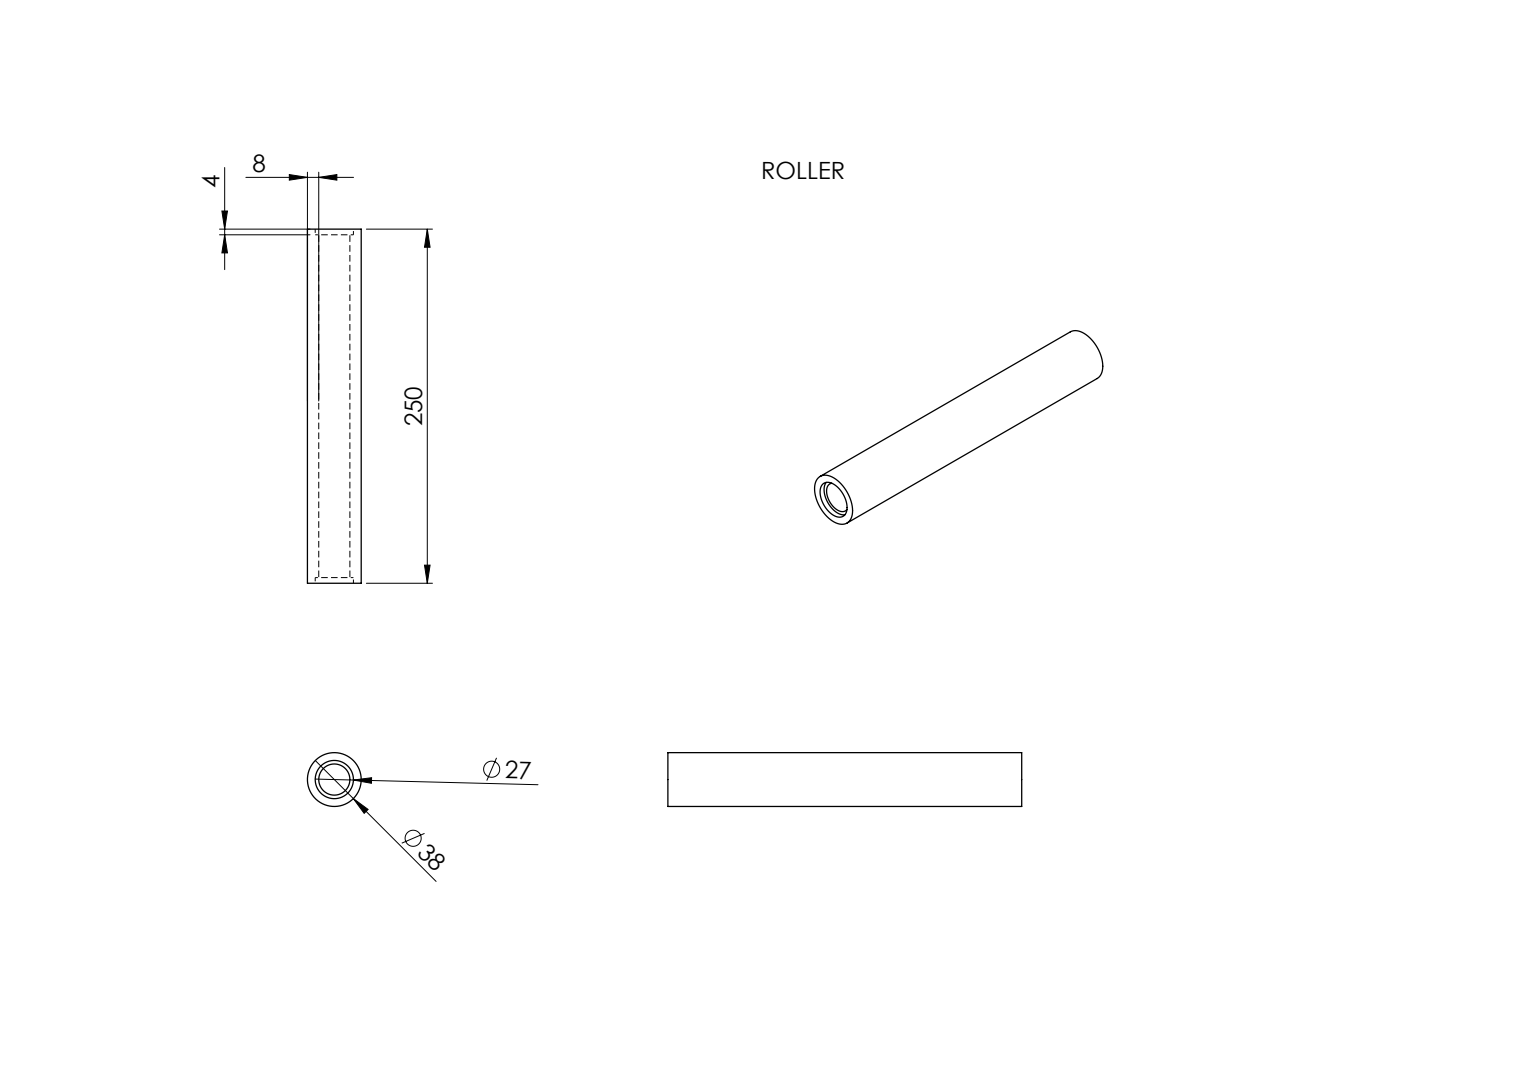
ISO-10303-21;
HEADER;
FILE_DESCRIPTION (('STEP AP214'),
    '1' );
FILE_NAME ('roller.step',
    '2026-10-24T14:05:44',
    ( '' ),
    ( '' ),
    'SwSTEP 2.0',
    'SolidWorks 2026',
    '' );
FILE_SCHEMA (( 'AUTOMOTIVE_DESIGN' ));
ENDSEC;

DATA;
#78=ADVANCED_FACE ( 'NONE', ( #707 ), #151, .F. ) ;
#101=CARTESIAN_POINT ( 'NONE',  ( 11.00000000000000000, 1.347111479062088405E-15, 121.0000000000000000 ) ) ;
#129=DIRECTION ( 'NONE',  ( 0.000000000000000000, 0.000000000000000000, 1.000000000000000000 ) ) ;
#130=DIRECTION ( 'NONE',  ( 0.000000000000000000, 0.000000000000000000, 1.000000000000000000 ) ) ;
#141=SURFACE_STYLE_USAGE ( .BOTH. , #4095 ) ;
#145=ADVANCED_FACE ( 'NONE', ( #6026 ), #5486, .F. ) ;
#151=CYLINDRICAL_SURFACE ( 'NONE', #6391, 13.50000000000000000 ) ;
#167=PLANE ( 'NONE',  #1333 ) ;
#204=ORIENTED_EDGE ( 'NONE', *, *, #2954, .T. ) ;
#232=EDGE_LOOP ( 'NONE', ( #859, #5751, #5107, #3402 ) ) ;
#286=EDGE_CURVE ( 'NONE', #7309, #3129, #6272, .T. ) ;
#299=CARTESIAN_POINT ( 'NONE',  ( 0.000000000000000000, 0.000000000000000000, 125.0000000000000000 ) ) ;
#385=DIRECTION ( 'NONE',  ( -0.000000000000000000, -0.000000000000000000, 1.000000000000000000 ) ) ;
#402=ADVANCED_BREP_SHAPE_REPRESENTATION ( '', ( #3126, #1963 ), #3131 ) ;
#447=AXIS2_PLACEMENT_3D ( 'NONE', #2275, #5736, #5768 ) ;
#495=CARTESIAN_POINT ( 'NONE',  ( 0.000000000000000000, 0.000000000000000000, -121.0000000000000000 ) ) ;
#501=EDGE_LOOP ( 'NONE', ( #2407, #5320, #3926, #4754 ) ) ;
#548=ORIENTED_EDGE ( 'NONE', *, *, #7125, .F. ) ;
#563=VERTEX_POINT ( 'NONE', #6568 ) ;
#566=CARTESIAN_POINT ( 'NONE',  ( -11.00000000000000000, 0.000000000000000000, 121.0000000000000000 ) ) ;
#628=DIRECTION ( 'NONE',  ( 0.000000000000000000, 0.000000000000000000, 1.000000000000000000 ) ) ;
#632=CIRCLE ( 'NONE', #7087, 19.00000000000000000 ) ;
#661=AXIS2_PLACEMENT_3D ( 'NONE', #7149, #4263, #2002 ) ;
#679=EDGE_LOOP ( 'NONE', ( #1531, #1316, #1080, #4303 ) ) ;
#681=DIRECTION ( 'NONE',  ( 1.000000000000000000, 0.000000000000000000, 0.000000000000000000 ) ) ;
#707=FACE_OUTER_BOUND ( 'NONE', #3501, .T. ) ;
#714=CARTESIAN_POINT ( 'NONE',  ( 0.000000000000000000, 0.000000000000000000, -121.0000000000000000 ) ) ;
#725=VECTOR ( 'NONE', #6797, 1000.000000000000000 ) ;
#761=ORIENTED_EDGE ( 'NONE', *, *, #5228, .T. ) ;
#764=AXIS2_PLACEMENT_3D ( 'NONE', #2213, #6804, #3945 ) ;
#780=AXIS2_PLACEMENT_3D ( 'NONE', #2339, #3531, #2993 ) ;
#787=DIRECTION ( 'NONE',  ( 1.000000000000000000, 0.000000000000000000, 0.000000000000000000 ) ) ;
#821=CARTESIAN_POINT ( 'NONE',  ( 0.000000000000000000, 0.000000000000000000, 125.0000000000000000 ) ) ;
#830=FACE_OUTER_BOUND ( 'NONE', #3358, .T. ) ;
#836=DIRECTION ( 'NONE',  ( -1.000000000000000000, 0.000000000000000000, 0.000000000000000000 ) ) ;
#859=ORIENTED_EDGE ( 'NONE', *, *, #4888, .F. ) ;
#866=AXIS2_PLACEMENT_3D ( 'NONE', #939, #3814, #4267 ) ;
#869=ORIENTED_EDGE ( 'NONE', *, *, #7028, .F. ) ;
#871=LINE ( 'NONE', #916, #4310 ) ;
#890=DIRECTION ( 'NONE',  ( -0.000000000000000000, -0.000000000000000000, -1.000000000000000000 ) ) ;
#902=ADVANCED_FACE ( 'NONE', ( #7143 ), #5410, .F. ) ;
#916=CARTESIAN_POINT ( 'NONE',  ( 13.50000000000000000, 1.653273178848926867E-15, -121.0000000000000000 ) ) ;
#921=AXIS2_PLACEMENT_3D ( 'NONE', #299, #2557, #3103 ) ;
#926=EDGE_CURVE ( 'NONE', #5946, #2821, #3721, .T. ) ;
#939=CARTESIAN_POINT ( 'NONE',  ( 0.000000000000000000, 0.000000000000000000, 125.0000000000000000 ) ) ;
#967=DIRECTION ( 'NONE',  ( 1.000000000000000000, 0.000000000000000000, 0.000000000000000000 ) ) ;
#993=DIRECTION ( 'NONE',  ( 0.000000000000000000, 0.000000000000000000, 1.000000000000000000 ) ) ;
#1017=DIRECTION ( 'NONE',  ( -0.000000000000000000, -0.000000000000000000, 1.000000000000000000 ) ) ;
#1022=CIRCLE ( 'NONE', #661, 11.00000000000000000 ) ;
#1027=PLANE ( 'NONE',  #4902 ) ;
#1029=CIRCLE ( 'NONE', #780, 19.00000000000000000 ) ;
#1044=ORIENTED_EDGE ( 'NONE', *, *, #286, .F. ) ;
#1063=DIRECTION ( 'NONE',  ( 1.000000000000000000, 0.000000000000000000, -0.000000000000000000 ) ) ;
#1069=CYLINDRICAL_SURFACE ( 'NONE', #764, 19.00000000000000000 ) ;
#1080=ORIENTED_EDGE ( 'NONE', *, *, #7028, .T. ) ;
#1133=CARTESIAN_POINT ( 'NONE',  ( 0.000000000000000000, 0.000000000000000000, 121.0000000000000000 ) ) ;
#1190=( NAMED_UNIT ( * ) PLANE_ANGLE_UNIT ( ) SI_UNIT ( $, .RADIAN. ) );
#1218=SHAPE_DEFINITION_REPRESENTATION ( #4339, #6025 ) ;
#1242=LINE ( 'NONE', #3584, #6951 ) ;
#1270=VECTOR ( 'NONE', #890, 1000.000000000000000 ) ;
#1277=FACE_OUTER_BOUND ( 'NONE', #3592, .T. ) ;
#1304=VERTEX_POINT ( 'NONE', #3677 ) ;
#1316=ORIENTED_EDGE ( 'NONE', *, *, #3473, .T. ) ;
#1333=AXIS2_PLACEMENT_3D ( 'NONE', #5931, #5284, #1979 ) ;
#1348=DIRECTION ( 'NONE',  ( -0.000000000000000000, -0.000000000000000000, -1.000000000000000000 ) ) ;
#1431=ORIENTED_EDGE ( 'NONE', *, *, #6454, .F. ) ;
#1463=DIRECTION ( 'NONE',  ( 1.000000000000000000, 0.000000000000000000, 0.000000000000000000 ) ) ;
#1531=ORIENTED_EDGE ( 'NONE', *, *, #3496, .F. ) ;
#1547=CARTESIAN_POINT ( 'NONE',  ( 0.000000000000000000, 0.000000000000000000, 121.0000000000000000 ) ) ;
#1551=CARTESIAN_POINT ( 'NONE',  ( 0.000000000000000000, 0.000000000000000000, 125.0000000000000000 ) ) ;
#1579=DIRECTION ( 'NONE',  ( 0.000000000000000000, 0.000000000000000000, 1.000000000000000000 ) ) ;
#1650=EDGE_CURVE ( 'NONE', #1304, #6651, #5323, .T. ) ;
#1673=AXIS2_PLACEMENT_3D ( 'NONE', #4611, #1579, #681 ) ;
#1693=EDGE_CURVE ( 'NONE', #2821, #2892, #6895, .T. ) ;
#1701=( NAMED_UNIT ( * ) PLANE_ANGLE_UNIT ( ) SI_UNIT ( $, .RADIAN. ) );
#1732=CIRCLE ( 'NONE', #3884, 13.50000000000000000 ) ;
#1741=AXIS2_PLACEMENT_3D ( 'NONE', #5744, #3477, #6877 ) ;
#1773=( NAMED_UNIT ( * ) SI_UNIT ( $, .STERADIAN. ) SOLID_ANGLE_UNIT ( ) );
#1804=AXIS2_PLACEMENT_3D ( 'NONE', #821, #6480, #1887 ) ;
#1840=EDGE_CURVE ( 'NONE', #5914, #2630, #6783, .T. ) ;
#1846=( LENGTH_UNIT ( ) NAMED_UNIT ( * ) SI_UNIT ( .MILLI., .METRE. ) );
#1854=DIRECTION ( 'NONE',  ( -0.000000000000000000, -0.000000000000000000, 1.000000000000000000 ) ) ;
#1880=ORIENTED_EDGE ( 'NONE', *, *, #6777, .F. ) ;
#1887=DIRECTION ( 'NONE',  ( 1.000000000000000000, 0.000000000000000000, 0.000000000000000000 ) ) ;
#1918=ORIENTED_EDGE ( 'NONE', *, *, #4537, .F. ) ;
#1927=ORIENTED_EDGE ( 'NONE', *, *, #5201, .F. ) ;
#1952=VECTOR ( 'NONE', #5276, 1000.000000000000000 ) ;
#1963=AXIS2_PLACEMENT_3D ( 'NONE', #2294, #628, #5829 ) ;
#1979=DIRECTION ( 'NONE',  ( 1.000000000000000000, 0.000000000000000000, 0.000000000000000000 ) ) ;
#2002=DIRECTION ( 'NONE',  ( 1.000000000000000000, 0.000000000000000000, 0.000000000000000000 ) ) ;
#2016=DIRECTION ( 'NONE',  ( 1.000000000000000000, 0.000000000000000000, -0.000000000000000000 ) ) ;
#2020=AXIS2_PLACEMENT_3D ( 'NONE', #2835, #4539, #2309 ) ;
#2068=EDGE_CURVE ( 'NONE', #5338, #4282, #6898, .T. ) ;
#2093=ORIENTED_EDGE ( 'NONE', *, *, #6554, .T. ) ;
#2169=DIRECTION ( 'NONE',  ( 1.000000000000000000, 0.000000000000000000, 0.000000000000000000 ) ) ;
#2213=CARTESIAN_POINT ( 'NONE',  ( 0.000000000000000000, 0.000000000000000000, 125.0000000000000000 ) ) ;
#2222=( NAMED_UNIT ( * ) SI_UNIT ( $, .STERADIAN. ) SOLID_ANGLE_UNIT ( ) );
#2239=ORIENTED_EDGE ( 'NONE', *, *, #1650, .F. ) ;
#2247=VERTEX_POINT ( 'NONE', #3350 ) ;
#2250=CYLINDRICAL_SURFACE ( 'NONE', #4673, 11.00000000000000000 ) ;
#2275=CARTESIAN_POINT ( 'NONE',  ( 0.000000000000000000, 0.000000000000000000, -121.0000000000000000 ) ) ;
#2294=CARTESIAN_POINT ( 'NONE',  ( 0.000000000000000000, 0.000000000000000000, 0.000000000000000000 ) ) ;
#2309=DIRECTION ( 'NONE',  ( 1.000000000000000000, 0.000000000000000000, 0.000000000000000000 ) ) ;
#2326=CIRCLE ( 'NONE', #3492, 11.00000000000000000 ) ;
#2332=ADVANCED_FACE ( 'NONE', ( #6011 ), #2543, .T. ) ;
#2339=CARTESIAN_POINT ( 'NONE',  ( 0.000000000000000000, 0.000000000000000000, -125.0000000000000000 ) ) ;
#2347=DIRECTION ( 'NONE',  ( -0.000000000000000000, -0.000000000000000000, 1.000000000000000000 ) ) ;
#2357=ORIENTED_EDGE ( 'NONE', *, *, #1650, .T. ) ;
#2363=FILL_AREA_STYLE_COLOUR ( '', #3752 ) ;
#2407=ORIENTED_EDGE ( 'NONE', *, *, #286, .T. ) ;
#2475=UNCERTAINTY_MEASURE_WITH_UNIT (LENGTH_MEASURE( 1.000000000000000082E-05 ), #1846, 'distance_accuracy_value', 'NONE');
#2492=VERTEX_POINT ( 'NONE', #3787 ) ;
#2532=LINE ( 'NONE', #7123, #4205 ) ;
#2540=( GEOMETRIC_REPRESENTATION_CONTEXT ( 3 ) GLOBAL_UNCERTAINTY_ASSIGNED_CONTEXT ( ( #2475 ) ) GLOBAL_UNIT_ASSIGNED_CONTEXT ( ( #1846, #3794, #3711 ) ) REPRESENTATION_CONTEXT ( 'NONE', 'WORKASPACE' ) );
#2543=CYLINDRICAL_SURFACE ( 'NONE', #3635, 19.00000000000000000 ) ;
#2557=DIRECTION ( 'NONE',  ( -0.000000000000000000, -0.000000000000000000, -1.000000000000000000 ) ) ;
#2590=ORIENTED_EDGE ( 'NONE', *, *, #1840, .F. ) ;
#2622=SHAPE_REPRESENTATION_RELATIONSHIP ( 'NONE' , 'NONE' ,  #6025, #402 ) ;
#2630=VERTEX_POINT ( 'NONE', #3981 ) ;
#2633=CARTESIAN_POINT ( 'NONE',  ( 0.000000000000000000, 0.000000000000000000, 121.0000000000000000 ) ) ;
#2643=CARTESIAN_POINT ( 'NONE',  ( 19.00000000000000000, 2.326828918379970970E-15, -125.0000000000000000 ) ) ;
#2692=ORIENTED_EDGE ( 'NONE', *, *, #5228, .F. ) ;
#2731=DIRECTION ( 'NONE',  ( -0.000000000000000000, -0.000000000000000000, 1.000000000000000000 ) ) ;
#2743=ADVANCED_FACE ( 'NONE', ( #5710 ), #1069, .T. ) ;
#2746=ORIENTED_EDGE ( 'NONE', *, *, #6777, .T. ) ;
#2799=ORIENTED_EDGE ( 'NONE', *, *, #3881, .F. ) ;
#2821=VERTEX_POINT ( 'NONE', #5925 ) ;
#2829=ADVANCED_FACE ( 'NONE', ( #5319, #1277 ), #6523, .F. ) ;
#2835=CARTESIAN_POINT ( 'NONE',  ( 0.000000000000000000, 0.000000000000000000, 125.0000000000000000 ) ) ;
#2877=CARTESIAN_POINT ( 'NONE',  ( -11.00000000000000000, 0.000000000000000000, -121.0000000000000000 ) ) ;
#2885=MECHANICAL_DESIGN_GEOMETRIC_PRESENTATION_REPRESENTATION('',(#6746),#6383);
#2892=VERTEX_POINT ( 'NONE', #2643 ) ;
#2909=CARTESIAN_POINT ( 'NONE',  ( 0.000000000000000000, 0.000000000000000000, -125.0000000000000000 ) ) ;
#2954=EDGE_CURVE ( 'NONE', #5946, #6812, #6261, .T. ) ;
#2968=LINE ( 'NONE', #3574, #1952 ) ;
#2993=DIRECTION ( 'NONE',  ( 1.000000000000000000, 0.000000000000000000, 0.000000000000000000 ) ) ;
#3011=EDGE_LOOP ( 'NONE', ( #1044, #5050 ) ) ;
#3048=ORIENTED_EDGE ( 'NONE', *, *, #6454, .T. ) ;
#3069=EDGE_LOOP ( 'NONE', ( #548, #4659 ) ) ;
#3087=FACE_BOUND ( 'NONE', #3069, .T. ) ;
#3095=ORIENTED_EDGE ( 'NONE', *, *, #3473, .F. ) ;
#3103=DIRECTION ( 'NONE',  ( -1.000000000000000000, 0.000000000000000000, 0.000000000000000000 ) ) ;
#3126=MANIFOLD_SOLID_BREP ( 'Mirror1', #3382 ) ;
#3129=VERTEX_POINT ( 'NONE', #101 ) ;
#3131=( GEOMETRIC_REPRESENTATION_CONTEXT ( 3 ) GLOBAL_UNCERTAINTY_ASSIGNED_CONTEXT ( ( #3600 ) ) GLOBAL_UNIT_ASSIGNED_CONTEXT ( ( #4741, #1190, #1773 ) ) REPRESENTATION_CONTEXT ( 'NONE', 'WORKASPACE' ) );
#3132=FACE_BOUND ( 'NONE', #3568, .T. ) ;
#3195=PRODUCT_DEFINITION ( 'UNKNOWN', '', #5539, #3735 ) ;
#3342=EDGE_LOOP ( 'NONE', ( #761, #2357 ) ) ;
#3350=CARTESIAN_POINT ( 'NONE',  ( 13.50000000000000000, 0.000000000000000000, 125.0000000000000000 ) ) ;
#3358=EDGE_LOOP ( 'NONE', ( #5719, #1880 ) ) ;
#3360=FACE_BOUND ( 'NONE', #3011, .T. ) ;
#3371=DIRECTION ( 'NONE',  ( -1.000000000000000000, 0.000000000000000000, 0.000000000000000000 ) ) ;
#3382=CLOSED_SHELL ( 'NONE', ( #7339, #145, #2743, #4663, #902, #4587, #2829, #2332, #78, #5151, #3724, #3467 ) ) ;
#3395=DIRECTION ( 'NONE',  ( 1.000000000000000000, 0.000000000000000000, 0.000000000000000000 ) ) ;
#3402=ORIENTED_EDGE ( 'NONE', *, *, #7125, .T. ) ;
#3406=CYLINDRICAL_SURFACE ( 'NONE', #4924, 13.50000000000000000 ) ;
#3420=( LENGTH_UNIT ( ) NAMED_UNIT ( * ) SI_UNIT ( .MILLI., .METRE. ) );
#3465=VECTOR ( 'NONE', #6057, 1000.000000000000000 ) ;
#3467=ADVANCED_FACE ( 'NONE', ( #3087, #830 ), #167, .T. ) ;
#3473=EDGE_CURVE ( 'NONE', #6812, #2892, #2532, .T. ) ;
#3477=DIRECTION ( 'NONE',  ( 0.000000000000000000, 0.000000000000000000, 1.000000000000000000 ) ) ;
#3492=AXIS2_PLACEMENT_3D ( 'NONE', #5371, #3767, #7176 ) ;
#3496=EDGE_CURVE ( 'NONE', #6812, #5946, #632, .T. ) ;
#3501=EDGE_LOOP ( 'NONE', ( #5742, #2692, #7036, #6067 ) ) ;
#3502=CARTESIAN_POINT ( 'NONE',  ( 11.00000000000000000, 1.347111479062088405E-15, -121.0000000000000000 ) ) ;
#3510=DIRECTION ( 'NONE',  ( 1.000000000000000000, 0.000000000000000000, -0.000000000000000000 ) ) ;
#3531=DIRECTION ( 'NONE',  ( 0.000000000000000000, 0.000000000000000000, 1.000000000000000000 ) ) ;
#3548=CARTESIAN_POINT ( 'NONE',  ( 0.000000000000000000, 0.000000000000000000, 121.0000000000000000 ) ) ;
#3568=EDGE_LOOP ( 'NONE', ( #1927, #2799 ) ) ;
#3574=CARTESIAN_POINT ( 'NONE',  ( -13.50000000000000000, 1.653273178848926867E-15, 121.0000000000000000 ) ) ;
#3584=CARTESIAN_POINT ( 'NONE',  ( 11.00000000000000000, 1.347111479062088405E-15, 125.0000000000000000 ) ) ;
#3592=EDGE_LOOP ( 'NONE', ( #5804, #869 ) ) ;
#3597=ORIENTED_EDGE ( 'NONE', *, *, #926, .T. ) ;
#3600=UNCERTAINTY_MEASURE_WITH_UNIT (LENGTH_MEASURE( 1.000000000000000082E-05 ), #4741, 'distance_accuracy_value', 'NONE');
#3635=AXIS2_PLACEMENT_3D ( 'NONE', #5973, #6498, #836 ) ;
#3641=AXIS2_PLACEMENT_3D ( 'NONE', #3548, #129, #6318 ) ;
#3677=CARTESIAN_POINT ( 'NONE',  ( -13.50000000000000000, 1.653273178848926867E-15, 121.0000000000000000 ) ) ;
#3683=DIRECTION ( 'NONE',  ( -0.000000000000000000, -0.000000000000000000, 1.000000000000000000 ) ) ;
#3694=CIRCLE ( 'NONE', #1673, 13.50000000000000000 ) ;
#3711=( NAMED_UNIT ( * ) SI_UNIT ( $, .STERADIAN. ) SOLID_ANGLE_UNIT ( ) );
#3721=LINE ( 'NONE', #6027, #1270 ) ;
#3724=ADVANCED_FACE ( 'NONE', ( #6866 ), #3406, .F. ) ;
#3735=PRODUCT_DEFINITION_CONTEXT ( 'detailed design', #4775, 'design' ) ;
#3752=COLOUR_RGB ( '',0.8941176470588234615, 0.8941176470588234615, 0.8941176470588234615 ) ;
#3755=ORIENTED_EDGE ( 'NONE', *, *, #1840, .T. ) ;
#3767=DIRECTION ( 'NONE',  ( 0.000000000000000000, 0.000000000000000000, -1.000000000000000000 ) ) ;
#3787=CARTESIAN_POINT ( 'NONE',  ( 13.50000000000000000, 1.653273178848926867E-15, -121.0000000000000000 ) ) ;
#3791=CARTESIAN_POINT ( 'NONE',  ( -11.00000000000000000, 0.000000000000000000, 125.0000000000000000 ) ) ;
#3794=( NAMED_UNIT ( * ) PLANE_ANGLE_UNIT ( ) SI_UNIT ( $, .RADIAN. ) );
#3814=DIRECTION ( 'NONE',  ( 0.000000000000000000, 0.000000000000000000, 1.000000000000000000 ) ) ;
#3819=DIRECTION ( 'NONE',  ( 1.000000000000000000, 0.000000000000000000, 0.000000000000000000 ) ) ;
#3859=LINE ( 'NONE', #6757, #725 ) ;
#3881=EDGE_CURVE ( 'NONE', #7016, #2247, #4451, .T. ) ;
#3884=AXIS2_PLACEMENT_3D ( 'NONE', #714, #2347, #787 ) ;
#3926=ORIENTED_EDGE ( 'NONE', *, *, #2068, .T. ) ;
#3945=DIRECTION ( 'NONE',  ( -1.000000000000000000, 0.000000000000000000, 0.000000000000000000 ) ) ;
#3952=CARTESIAN_POINT ( 'NONE',  ( 13.50000000000000000, 1.653273178848926867E-15, -125.0000000000000000 ) ) ;
#3963=AXIS2_PLACEMENT_3D ( 'NONE', #1551, #993, #2016 ) ;
#3981=CARTESIAN_POINT ( 'NONE',  ( -13.50000000000000000, 0.000000000000000000, -125.0000000000000000 ) ) ;
#4070=ORIENTED_EDGE ( 'NONE', *, *, #6559, .T. ) ;
#4095=SURFACE_SIDE_STYLE ('',( #6950 ) ) ;
#4144=DIRECTION ( 'NONE',  ( 1.000000000000000000, 0.000000000000000000, 0.000000000000000000 ) ) ;
#4173=ORIENTED_EDGE ( 'NONE', *, *, #5103, .F. ) ;
#4205=VECTOR ( 'NONE', #1348, 1000.000000000000000 ) ;
#4263=DIRECTION ( 'NONE',  ( 0.000000000000000000, 0.000000000000000000, 1.000000000000000000 ) ) ;
#4267=DIRECTION ( 'NONE',  ( 1.000000000000000000, 0.000000000000000000, 0.000000000000000000 ) ) ;
#4272=CARTESIAN_POINT ( 'NONE',  ( 0.000000000000000000, 0.000000000000000000, 125.0000000000000000 ) ) ;
#4282=VERTEX_POINT ( 'NONE', #2877 ) ;
#4303=ORIENTED_EDGE ( 'NONE', *, *, #926, .F. ) ;
#4310=VECTOR ( 'NONE', #7129, 1000.000000000000000 ) ;
#4339=PRODUCT_DEFINITION_SHAPE ( 'NONE', 'NONE',  #3195 ) ;
#4370=AXIS2_PLACEMENT_3D ( 'NONE', #495, #1017, #3395 ) ;
#4419=CARTESIAN_POINT ( 'NONE',  ( 13.50000000000000000, 0.000000000000000000, 121.0000000000000000 ) ) ;
#4446=CYLINDRICAL_SURFACE ( 'NONE', #5807, 13.50000000000000000 ) ;
#4451=CIRCLE ( 'NONE', #1804, 13.50000000000000000 ) ;
#4537=EDGE_CURVE ( 'NONE', #2492, #5914, #871, .T. ) ;
#4539=DIRECTION ( 'NONE',  ( 0.000000000000000000, 0.000000000000000000, 1.000000000000000000 ) ) ;
#4541=DIRECTION ( 'NONE',  ( -1.000000000000000000, 0.000000000000000000, 0.000000000000000000 ) ) ;
#4547=FACE_OUTER_BOUND ( 'NONE', #501, .T. ) ;
#4576=EDGE_CURVE ( 'NONE', #7309, #4282, #5436, .T. ) ;
#4587=ADVANCED_FACE ( 'NONE', ( #3132, #7164 ), #4839, .T. ) ;
#4607=CIRCLE ( 'NONE', #6292, 13.50000000000000000 ) ;
#4611=CARTESIAN_POINT ( 'NONE',  ( 0.000000000000000000, 0.000000000000000000, 121.0000000000000000 ) ) ;
#4638=EDGE_LOOP ( 'NONE', ( #2093, #7180, #1431, #4173 ) ) ;
#4659=ORIENTED_EDGE ( 'NONE', *, *, #2068, .F. ) ;
#4663=ADVANCED_FACE ( 'NONE', ( #4547 ), #2250, .F. ) ;
#4673=AXIS2_PLACEMENT_3D ( 'NONE', #5670, #6207, #3371 ) ;
#4681=UNCERTAINTY_MEASURE_WITH_UNIT (LENGTH_MEASURE( 1.000000000000000082E-05 ), #3420, 'distance_accuracy_value', 'NONE');
#4709=CARTESIAN_POINT ( 'NONE',  ( 0.000000000000000000, 0.000000000000000000, 121.0000000000000000 ) ) ;
#4741=( LENGTH_UNIT ( ) NAMED_UNIT ( * ) SI_UNIT ( .MILLI., .METRE. ) );
#4754=ORIENTED_EDGE ( 'NONE', *, *, #4576, .F. ) ;
#4775=APPLICATION_CONTEXT ( 'automotive_design' ) ;
#4839=PLANE ( 'NONE',  #3963 ) ;
#4888=EDGE_CURVE ( 'NONE', #3129, #5338, #1242, .T. ) ;
#4902=AXIS2_PLACEMENT_3D ( 'NONE', #1133, #5657, #1063 ) ;
#4903=ORIENTED_EDGE ( 'NONE', *, *, #5038, .F. ) ;
#4906=CARTESIAN_POINT ( 'NONE',  ( 13.50000000000000000, 0.000000000000000000, 121.0000000000000000 ) ) ;
#4919=ORIENTED_EDGE ( 'NONE', *, *, #3881, .T. ) ;
#4924=AXIS2_PLACEMENT_3D ( 'NONE', #6833, #5079, #4541 ) ;
#5029=FACE_OUTER_BOUND ( 'NONE', #3342, .T. ) ;
#5038=EDGE_CURVE ( 'NONE', #6651, #2247, #5500, .T. ) ;
#5050=ORIENTED_EDGE ( 'NONE', *, *, #6689, .F. ) ;
#5079=DIRECTION ( 'NONE',  ( -0.000000000000000000, -0.000000000000000000, -1.000000000000000000 ) ) ;
#5080=AXIS2_PLACEMENT_3D ( 'NONE', #1547, #6203, #1463 ) ;
#5103=EDGE_CURVE ( 'NONE', #563, #2630, #3859, .T. ) ;
#5107=ORIENTED_EDGE ( 'NONE', *, *, #4576, .T. ) ;
#5115=ORIENTED_EDGE ( 'NONE', *, *, #1693, .T. ) ;
#5151=ADVANCED_FACE ( 'NONE', ( #3360, #5029 ), #1027, .T. ) ;
#5201=EDGE_CURVE ( 'NONE', #2247, #7016, #5260, .T. ) ;
#5228=EDGE_CURVE ( 'NONE', #6651, #1304, #3694, .T. ) ;
#5232=CARTESIAN_POINT ( 'NONE',  ( -13.50000000000000000, 1.653273178848926867E-15, 125.0000000000000000 ) ) ;
#5260=CIRCLE ( 'NONE', #2020, 13.50000000000000000 ) ;
#5276=DIRECTION ( 'NONE',  ( -0.000000000000000000, -0.000000000000000000, 1.000000000000000000 ) ) ;
#5284=DIRECTION ( 'NONE',  ( 0.000000000000000000, 0.000000000000000000, -1.000000000000000000 ) ) ;
#5285=CARTESIAN_POINT ( 'NONE',  ( -19.00000000000000000, 0.000000000000000000, 125.0000000000000000 ) ) ;
#5289=PRODUCT ( 'roller', 'roller', '', ( #6246 ) ) ;
#5319=FACE_BOUND ( 'NONE', #6524, .T. ) ;
#5320=ORIENTED_EDGE ( 'NONE', *, *, #4888, .T. ) ;
#5323=CIRCLE ( 'NONE', #3641, 13.50000000000000000 ) ;
#5325=DIRECTION ( 'NONE',  ( 1.000000000000000000, 0.000000000000000000, 0.000000000000000000 ) ) ;
#5338=VERTEX_POINT ( 'NONE', #3502 ) ;
#5371=CARTESIAN_POINT ( 'NONE',  ( 0.000000000000000000, 0.000000000000000000, -121.0000000000000000 ) ) ;
#5410=CYLINDRICAL_SURFACE ( 'NONE', #921, 11.00000000000000000 ) ;
#5436=LINE ( 'NONE', #3791, #3465 ) ;
#5486=CYLINDRICAL_SURFACE ( 'NONE', #7097, 13.50000000000000000 ) ;
#5500=LINE ( 'NONE', #4906, #6233 ) ;
#5501=CARTESIAN_POINT ( 'NONE',  ( 0.000000000000000000, 0.000000000000000000, -125.0000000000000000 ) ) ;
#5539=PRODUCT_DEFINITION_FORMATION_WITH_SPECIFIED_SOURCE ( 'ANY', '', #5289, .NOT_KNOWN. ) ;
#5558=MECHANICAL_DESIGN_GEOMETRIC_PRESENTATION_REPRESENTATION('',(#6516),#2540);
#5571=FACE_OUTER_BOUND ( 'NONE', #4638, .T. ) ;
#5584=ORIENTED_EDGE ( 'NONE', *, *, #2954, .F. ) ;
#5616=EDGE_LOOP ( 'NONE', ( #2239, #4070, #4919, #4903 ) ) ;
#5643=CARTESIAN_POINT ( 'NONE',  ( 0.000000000000000000, 0.000000000000000000, -121.0000000000000000 ) ) ;
#5657=DIRECTION ( 'NONE',  ( 0.000000000000000000, 0.000000000000000000, 1.000000000000000000 ) ) ;
#5670=CARTESIAN_POINT ( 'NONE',  ( 0.000000000000000000, 0.000000000000000000, 125.0000000000000000 ) ) ;
#5710=FACE_OUTER_BOUND ( 'NONE', #679, .T. ) ;
#5719=ORIENTED_EDGE ( 'NONE', *, *, #6554, .F. ) ;
#5736=DIRECTION ( 'NONE',  ( 0.000000000000000000, 0.000000000000000000, -1.000000000000000000 ) ) ;
#5742=ORIENTED_EDGE ( 'NONE', *, *, #6559, .F. ) ;
#5744=CARTESIAN_POINT ( 'NONE',  ( 0.000000000000000000, 0.000000000000000000, -125.0000000000000000 ) ) ;
#5751=ORIENTED_EDGE ( 'NONE', *, *, #6689, .T. ) ;
#5768=DIRECTION ( 'NONE',  ( -1.000000000000000000, 0.000000000000000000, 0.000000000000000000 ) ) ;
#5804=ORIENTED_EDGE ( 'NONE', *, *, #1693, .F. ) ;
#5807=AXIS2_PLACEMENT_3D ( 'NONE', #5643, #6138, #6702 ) ;
#5829=DIRECTION ( 'NONE',  ( 1.000000000000000000, 0.000000000000000000, 0.000000000000000000 ) ) ;
#5914=VERTEX_POINT ( 'NONE', #3952 ) ;
#5925=CARTESIAN_POINT ( 'NONE',  ( -19.00000000000000000, 0.000000000000000000, -125.0000000000000000 ) ) ;
#5931=CARTESIAN_POINT ( 'NONE',  ( 0.000000000000000000, 0.000000000000000000, -121.0000000000000000 ) ) ;
#5946=VERTEX_POINT ( 'NONE', #5285 ) ;
#5973=CARTESIAN_POINT ( 'NONE',  ( 0.000000000000000000, 0.000000000000000000, 125.0000000000000000 ) ) ;
#6011=FACE_OUTER_BOUND ( 'NONE', #6393, .T. ) ;
#6025=SHAPE_REPRESENTATION ( 'roller', ( #1963 ), #3131 ) ;
#6026=FACE_OUTER_BOUND ( 'NONE', #5616, .T. ) ;
#6027=CARTESIAN_POINT ( 'NONE',  ( -19.00000000000000000, 0.000000000000000000, 125.0000000000000000 ) ) ;
#6057=DIRECTION ( 'NONE',  ( -0.000000000000000000, -0.000000000000000000, -1.000000000000000000 ) ) ;
#6067=ORIENTED_EDGE ( 'NONE', *, *, #5201, .T. ) ;
#6138=DIRECTION ( 'NONE',  ( -0.000000000000000000, -0.000000000000000000, -1.000000000000000000 ) ) ;
#6203=DIRECTION ( 'NONE',  ( 0.000000000000000000, 0.000000000000000000, 1.000000000000000000 ) ) ;
#6207=DIRECTION ( 'NONE',  ( -0.000000000000000000, -0.000000000000000000, -1.000000000000000000 ) ) ;
#6233=VECTOR ( 'NONE', #385, 1000.000000000000000 ) ;
#6246=PRODUCT_CONTEXT ( 'NONE', #7329, 'mechanical' ) ;
#6261=CIRCLE ( 'NONE', #866, 19.00000000000000000 ) ;
#6272=CIRCLE ( 'NONE', #5080, 11.00000000000000000 ) ;
#6292=AXIS2_PLACEMENT_3D ( 'NONE', #6834, #6867, #2169 ) ;
#6318=DIRECTION ( 'NONE',  ( 1.000000000000000000, 0.000000000000000000, 0.000000000000000000 ) ) ;
#6383=( GEOMETRIC_REPRESENTATION_CONTEXT ( 3 ) GLOBAL_UNCERTAINTY_ASSIGNED_CONTEXT ( ( #4681 ) ) GLOBAL_UNIT_ASSIGNED_CONTEXT ( ( #3420, #1701, #2222 ) ) REPRESENTATION_CONTEXT ( 'NONE', 'WORKASPACE' ) );
#6391=AXIS2_PLACEMENT_3D ( 'NONE', #4709, #1854, #4144 ) ;
#6393=EDGE_LOOP ( 'NONE', ( #3095, #5584, #3597, #5115 ) ) ;
#6394=PRESENTATION_STYLE_ASSIGNMENT (( #141 ) ) ;
#6454=EDGE_CURVE ( 'NONE', #2630, #5914, #4607, .T. ) ;
#6480=DIRECTION ( 'NONE',  ( 0.000000000000000000, 0.000000000000000000, 1.000000000000000000 ) ) ;
#6498=DIRECTION ( 'NONE',  ( -0.000000000000000000, -0.000000000000000000, -1.000000000000000000 ) ) ;
#6516=STYLED_ITEM ( 'NONE', ( #6394 ), #402 ) ;
#6523=PLANE ( 'NONE',  #7094 ) ;
#6524=EDGE_LOOP ( 'NONE', ( #3048, #3755 ) ) ;
#6527=DIRECTION ( 'NONE',  ( -0.000000000000000000, -0.000000000000000000, -1.000000000000000000 ) ) ;
#6554=EDGE_CURVE ( 'NONE', #563, #2492, #1732, .T. ) ;
#6559=EDGE_CURVE ( 'NONE', #1304, #7016, #2968, .T. ) ;
#6568=CARTESIAN_POINT ( 'NONE',  ( -13.50000000000000000, 0.000000000000000000, -121.0000000000000000 ) ) ;
#6594=ORIENTED_EDGE ( 'NONE', *, *, #5103, .T. ) ;
#6642=CIRCLE ( 'NONE', #4370, 13.50000000000000000 ) ;
#6651=VERTEX_POINT ( 'NONE', #4419 ) ;
#6658=AXIS2_PLACEMENT_3D ( 'NONE', #5501, #2731, #3819 ) ;
#6689=EDGE_CURVE ( 'NONE', #3129, #7309, #1022, .T. ) ;
#6698=ORIENTED_EDGE ( 'NONE', *, *, #3496, .T. ) ;
#6702=DIRECTION ( 'NONE',  ( -1.000000000000000000, 0.000000000000000000, 0.000000000000000000 ) ) ;
#6746=STYLED_ITEM('',(#7432),#3126);
#6757=CARTESIAN_POINT ( 'NONE',  ( -13.50000000000000000, 0.000000000000000000, -121.0000000000000000 ) ) ;
#6777=EDGE_CURVE ( 'NONE', #2492, #563, #6642, .T. ) ;
#6783=CIRCLE ( 'NONE', #6658, 13.50000000000000000 ) ;
#6788=CARTESIAN_POINT ( 'NONE',  ( 19.00000000000000000, 2.326828918379970970E-15, 125.0000000000000000 ) ) ;
#6797=DIRECTION ( 'NONE',  ( -0.000000000000000000, -0.000000000000000000, -1.000000000000000000 ) ) ;
#6804=DIRECTION ( 'NONE',  ( -0.000000000000000000, -0.000000000000000000, -1.000000000000000000 ) ) ;
#6812=VERTEX_POINT ( 'NONE', #6788 ) ;
#6820=EDGE_LOOP ( 'NONE', ( #204, #6698 ) ) ;
#6833=CARTESIAN_POINT ( 'NONE',  ( 0.000000000000000000, 0.000000000000000000, -121.0000000000000000 ) ) ;
#6834=CARTESIAN_POINT ( 'NONE',  ( 0.000000000000000000, 0.000000000000000000, -125.0000000000000000 ) ) ;
#6866=FACE_OUTER_BOUND ( 'NONE', #7212, .T. ) ;
#6867=DIRECTION ( 'NONE',  ( -0.000000000000000000, -0.000000000000000000, 1.000000000000000000 ) ) ;
#6877=DIRECTION ( 'NONE',  ( 1.000000000000000000, 0.000000000000000000, 0.000000000000000000 ) ) ;
#6895=CIRCLE ( 'NONE', #1741, 19.00000000000000000 ) ;
#6898=CIRCLE ( 'NONE', #447, 11.00000000000000000 ) ;
#6936=DIRECTION ( 'NONE',  ( 0.000000000000000000, 0.000000000000000000, 1.000000000000000000 ) ) ;
#6950=SURFACE_STYLE_FILL_AREA ( #6989 ) ;
#6951=VECTOR ( 'NONE', #6527, 1000.000000000000000 ) ;
#6989=FILL_AREA_STYLE ('',( #2363 ) ) ;
#7016=VERTEX_POINT ( 'NONE', #5232 ) ;
#7028=EDGE_CURVE ( 'NONE', #2892, #2821, #1029, .T. ) ;
#7036=ORIENTED_EDGE ( 'NONE', *, *, #5038, .T. ) ;
#7087=AXIS2_PLACEMENT_3D ( 'NONE', #4272, #130, #5325 ) ;
#7094=AXIS2_PLACEMENT_3D ( 'NONE', #2909, #6936, #3510 ) ;
#7097=AXIS2_PLACEMENT_3D ( 'NONE', #2633, #3683, #967 ) ;
#7123=CARTESIAN_POINT ( 'NONE',  ( 19.00000000000000000, 2.326828918379970970E-15, 125.0000000000000000 ) ) ;
#7125=EDGE_CURVE ( 'NONE', #4282, #5338, #2326, .T. ) ;
#7129=DIRECTION ( 'NONE',  ( -0.000000000000000000, -0.000000000000000000, -1.000000000000000000 ) ) ;
#7143=FACE_OUTER_BOUND ( 'NONE', #232, .T. ) ;
#7149=CARTESIAN_POINT ( 'NONE',  ( 0.000000000000000000, 0.000000000000000000, 121.0000000000000000 ) ) ;
#7164=FACE_OUTER_BOUND ( 'NONE', #6820, .T. ) ;
#7176=DIRECTION ( 'NONE',  ( -1.000000000000000000, 0.000000000000000000, 0.000000000000000000 ) ) ;
#7180=ORIENTED_EDGE ( 'NONE', *, *, #4537, .T. ) ;
#7212=EDGE_LOOP ( 'NONE', ( #1918, #2746, #6594, #2590 ) ) ;
#7309=VERTEX_POINT ( 'NONE', #566 ) ;
#7329=APPLICATION_CONTEXT ( 'automotive_design' ) ;
#7339=ADVANCED_FACE ( 'NONE', ( #5571 ), #4446, .F. ) ;
#7426=COLOUR_RGB('Sky Blue',0.24,0.69,0.87);
#7427=FILL_AREA_STYLE_COLOUR('',#7426);
#7428=FILL_AREA_STYLE('',(#7427));
#7429=SURFACE_STYLE_FILL_AREA(#7428);
#7430=SURFACE_SIDE_STYLE('',(#7429));
#7431=SURFACE_STYLE_USAGE(.BOTH.,#7430);
#7432=PRESENTATION_STYLE_ASSIGNMENT((#7431));
ENDSEC;
END-ISO-10303-21;
